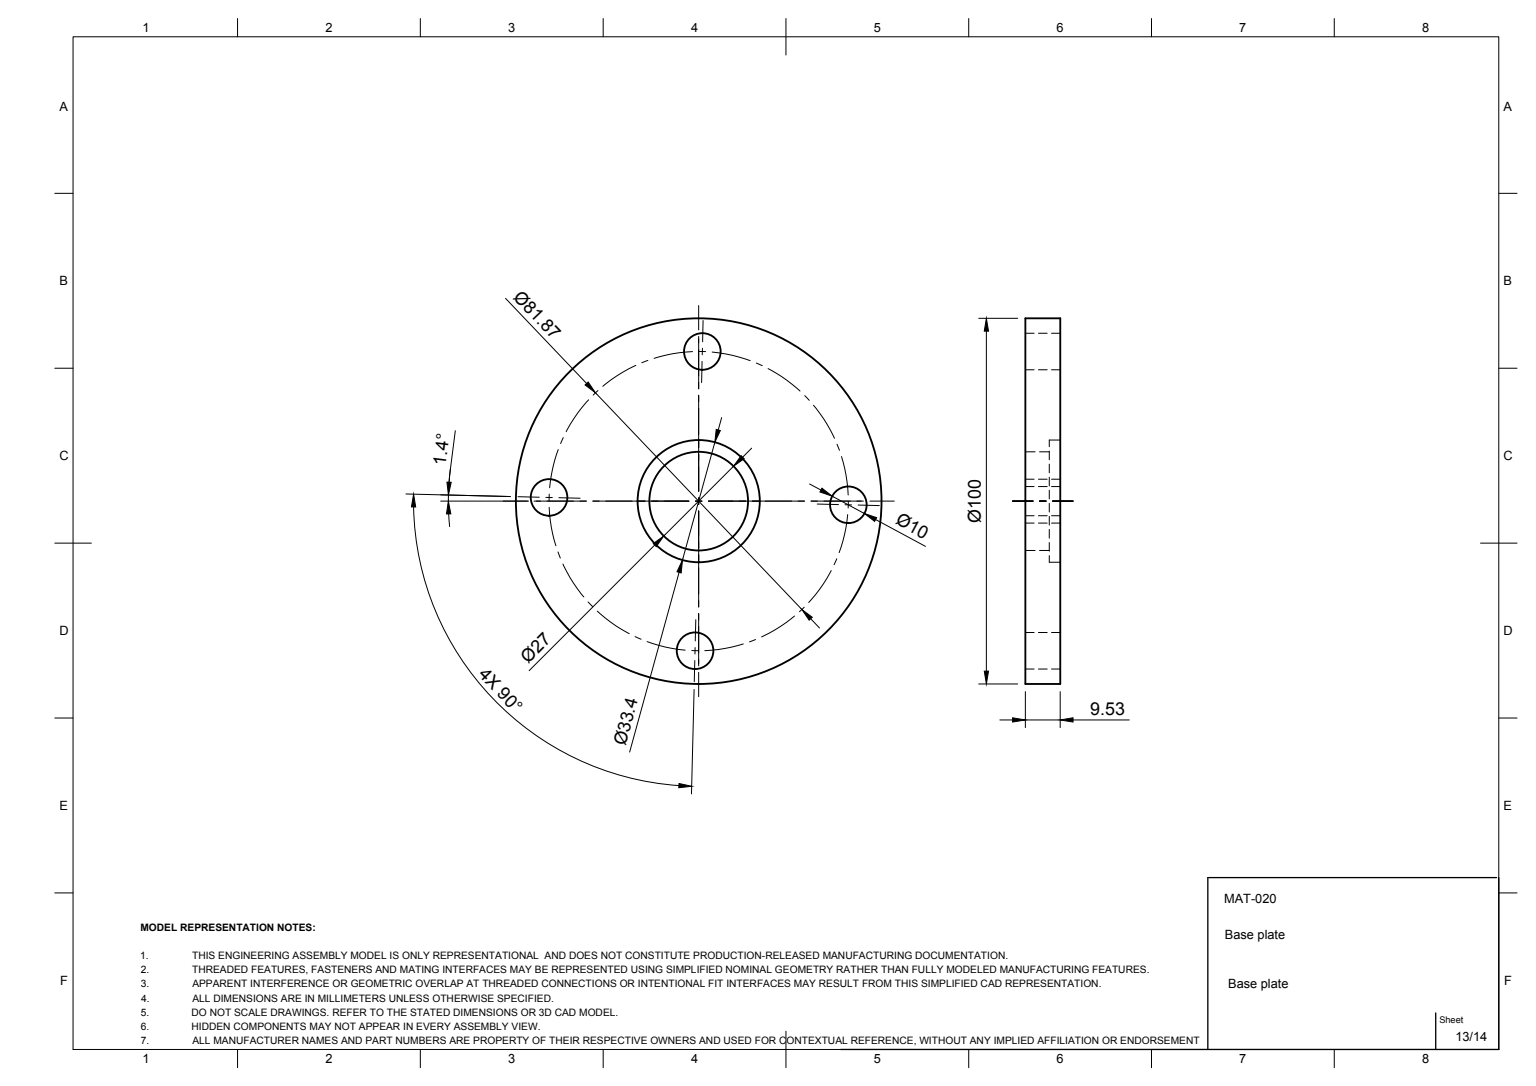
ISO-10303-21;
HEADER;
/* Generated by software containing ST-Developer
 * from STEP Tools, Inc. (www.steptools.com) 
 */

FILE_DESCRIPTION(
/* description */ ('STEP AP214'),
/* implementation_level */ '2;1');

FILE_NAME(
/* name */ 'Base Plate.step',
/* time_stamp */ '2026-11-14T06:20:50-08:00',
/* author */ (''),
/* organization */ (''),
/* preprocessor_version */ 'ST-DEVELOPER v20.2',
/* originating_system */ 'Autodesk Translation Framework v15.17.0.0',
/* authorisation */ '');

FILE_SCHEMA (('AUTOMOTIVE_DESIGN { 1 0 10303 214 3 1 1 }'));
ENDSEC;

DATA;
#10=MECHANICAL_DESIGN_GEOMETRIC_PRESENTATION_REPRESENTATION('',(#964),#20658);
#136=FACE_BOUND('',#1366,.T.);
#137=FACE_BOUND('',#1367,.T.);
#138=FACE_BOUND('',#1368,.T.);
#139=FACE_BOUND('',#1369,.T.);
#140=FACE_BOUND('',#1370,.T.);
#141=FACE_BOUND('',#1372,.T.);
#142=FACE_BOUND('',#1373,.T.);
#143=FACE_BOUND('',#1374,.T.);
#144=FACE_BOUND('',#1375,.T.);
#145=FACE_BOUND('',#1376,.T.);
#146=FACE_BOUND('',#1378,.T.);
#428=PLANE('',#4012);
#429=PLANE('',#4013);
#430=PLANE('',#4014);
#597=LINE('',#20343,#790);
#598=LINE('',#20349,#791);
#599=LINE('',#20355,#792);
#600=LINE('',#20361,#793);
#601=LINE('',#20367,#794);
#602=LINE('',#20373,#795);
#603=LINE('',#20379,#796);
#790=VECTOR('',#4672,13.5);
#791=VECTOR('',#4679,16.7);
#792=VECTOR('',#4686,5.);
#793=VECTOR('',#4693,5.);
#794=VECTOR('',#4700,5.);
#795=VECTOR('',#4707,5.);
#796=VECTOR('',#4714,50.);
#910=CYLINDRICAL_SURFACE('',#3991,13.5);
#911=CYLINDRICAL_SURFACE('',#3994,16.7);
#912=CYLINDRICAL_SURFACE('',#3997,5.);
#913=CYLINDRICAL_SURFACE('',#4000,5.);
#914=CYLINDRICAL_SURFACE('',#4003,5.);
#915=CYLINDRICAL_SURFACE('',#4006,5.);
#916=CYLINDRICAL_SURFACE('',#4009,50.);
#940=SHAPE_REPRESENTATION_RELATIONSHIP('SRR','None',#20724,#952);
#952=ADVANCED_BREP_SHAPE_REPRESENTATION('',(#976),#20654);
#964=STYLED_ITEM('',(#20788),#976);
#976=MANIFOLD_SOLID_BREP('Body1',#3659);
#1137=FACE_OUTER_BOUND('',#1358,.T.);
#1138=FACE_OUTER_BOUND('',#1359,.T.);
#1139=FACE_OUTER_BOUND('',#1360,.T.);
#1140=FACE_OUTER_BOUND('',#1361,.T.);
#1141=FACE_OUTER_BOUND('',#1362,.T.);
#1142=FACE_OUTER_BOUND('',#1363,.T.);
#1143=FACE_OUTER_BOUND('',#1364,.T.);
#1144=FACE_OUTER_BOUND('',#1365,.T.);
#1145=FACE_OUTER_BOUND('',#1371,.T.);
#1146=FACE_OUTER_BOUND('',#1377,.T.);
#1358=EDGE_LOOP('',(#3230,#3231,#3232,#3233));
#1359=EDGE_LOOP('',(#3234,#3235,#3236,#3237));
#1360=EDGE_LOOP('',(#3238,#3239,#3240,#3241));
#1361=EDGE_LOOP('',(#3242,#3243,#3244,#3245));
#1362=EDGE_LOOP('',(#3246,#3247,#3248,#3249));
#1363=EDGE_LOOP('',(#3250,#3251,#3252,#3253));
#1364=EDGE_LOOP('',(#3254,#3255,#3256,#3257));
#1365=EDGE_LOOP('',(#3258));
#1366=EDGE_LOOP('',(#3259));
#1367=EDGE_LOOP('',(#3260));
#1368=EDGE_LOOP('',(#3261));
#1369=EDGE_LOOP('',(#3262));
#1370=EDGE_LOOP('',(#3263));
#1371=EDGE_LOOP('',(#3264));
#1372=EDGE_LOOP('',(#3265));
#1373=EDGE_LOOP('',(#3266));
#1374=EDGE_LOOP('',(#3267));
#1375=EDGE_LOOP('',(#3268));
#1376=EDGE_LOOP('',(#3269));
#1377=EDGE_LOOP('',(#3270));
#1378=EDGE_LOOP('',(#3271));
#1493=CIRCLE('',#3992,13.5);
#1494=CIRCLE('',#3993,13.5);
#1495=CIRCLE('',#3995,16.7);
#1496=CIRCLE('',#3996,16.7);
#1497=CIRCLE('',#3998,5.);
#1498=CIRCLE('',#3999,5.);
#1499=CIRCLE('',#4001,5.);
#1500=CIRCLE('',#4002,5.);
#1501=CIRCLE('',#4004,5.);
#1502=CIRCLE('',#4005,5.);
#1503=CIRCLE('',#4007,5.);
#1504=CIRCLE('',#4008,5.);
#1505=CIRCLE('',#4010,50.);
#1506=CIRCLE('',#4011,50.);
#1821=VERTEX_POINT('',#20340);
#1822=VERTEX_POINT('',#20342);
#1823=VERTEX_POINT('',#20346);
#1824=VERTEX_POINT('',#20348);
#1825=VERTEX_POINT('',#20352);
#1826=VERTEX_POINT('',#20354);
#1827=VERTEX_POINT('',#20358);
#1828=VERTEX_POINT('',#20360);
#1829=VERTEX_POINT('',#20364);
#1830=VERTEX_POINT('',#20366);
#1831=VERTEX_POINT('',#20370);
#1832=VERTEX_POINT('',#20372);
#1833=VERTEX_POINT('',#20376);
#1834=VERTEX_POINT('',#20378);
#2297=EDGE_CURVE('',#1821,#1821,#1493,.T.);
#2298=EDGE_CURVE('',#1821,#1822,#597,.T.);
#2299=EDGE_CURVE('',#1822,#1822,#1494,.T.);
#2300=EDGE_CURVE('',#1823,#1823,#1495,.T.);
#2301=EDGE_CURVE('',#1823,#1824,#598,.T.);
#2302=EDGE_CURVE('',#1824,#1824,#1496,.T.);
#2303=EDGE_CURVE('',#1825,#1825,#1497,.T.);
#2304=EDGE_CURVE('',#1825,#1826,#599,.T.);
#2305=EDGE_CURVE('',#1826,#1826,#1498,.T.);
#2306=EDGE_CURVE('',#1827,#1827,#1499,.T.);
#2307=EDGE_CURVE('',#1827,#1828,#600,.T.);
#2308=EDGE_CURVE('',#1828,#1828,#1500,.T.);
#2309=EDGE_CURVE('',#1829,#1829,#1501,.T.);
#2310=EDGE_CURVE('',#1829,#1830,#601,.T.);
#2311=EDGE_CURVE('',#1830,#1830,#1502,.T.);
#2312=EDGE_CURVE('',#1831,#1831,#1503,.T.);
#2313=EDGE_CURVE('',#1831,#1832,#602,.T.);
#2314=EDGE_CURVE('',#1832,#1832,#1504,.T.);
#2315=EDGE_CURVE('',#1833,#1833,#1505,.T.);
#2316=EDGE_CURVE('',#1833,#1834,#603,.T.);
#2317=EDGE_CURVE('',#1834,#1834,#1506,.T.);
#3230=ORIENTED_EDGE('',*,*,#2297,.F.);
#3231=ORIENTED_EDGE('',*,*,#2298,.T.);
#3232=ORIENTED_EDGE('',*,*,#2299,.T.);
#3233=ORIENTED_EDGE('',*,*,#2298,.F.);
#3234=ORIENTED_EDGE('',*,*,#2300,.F.);
#3235=ORIENTED_EDGE('',*,*,#2301,.T.);
#3236=ORIENTED_EDGE('',*,*,#2302,.T.);
#3237=ORIENTED_EDGE('',*,*,#2301,.F.);
#3238=ORIENTED_EDGE('',*,*,#2303,.T.);
#3239=ORIENTED_EDGE('',*,*,#2304,.T.);
#3240=ORIENTED_EDGE('',*,*,#2305,.F.);
#3241=ORIENTED_EDGE('',*,*,#2304,.F.);
#3242=ORIENTED_EDGE('',*,*,#2306,.T.);
#3243=ORIENTED_EDGE('',*,*,#2307,.T.);
#3244=ORIENTED_EDGE('',*,*,#2308,.F.);
#3245=ORIENTED_EDGE('',*,*,#2307,.F.);
#3246=ORIENTED_EDGE('',*,*,#2309,.T.);
#3247=ORIENTED_EDGE('',*,*,#2310,.T.);
#3248=ORIENTED_EDGE('',*,*,#2311,.F.);
#3249=ORIENTED_EDGE('',*,*,#2310,.F.);
#3250=ORIENTED_EDGE('',*,*,#2312,.T.);
#3251=ORIENTED_EDGE('',*,*,#2313,.T.);
#3252=ORIENTED_EDGE('',*,*,#2314,.F.);
#3253=ORIENTED_EDGE('',*,*,#2313,.F.);
#3254=ORIENTED_EDGE('',*,*,#2315,.T.);
#3255=ORIENTED_EDGE('',*,*,#2316,.T.);
#3256=ORIENTED_EDGE('',*,*,#2317,.F.);
#3257=ORIENTED_EDGE('',*,*,#2316,.F.);
#3258=ORIENTED_EDGE('',*,*,#2317,.T.);
#3259=ORIENTED_EDGE('',*,*,#2309,.F.);
#3260=ORIENTED_EDGE('',*,*,#2303,.F.);
#3261=ORIENTED_EDGE('',*,*,#2302,.F.);
#3262=ORIENTED_EDGE('',*,*,#2306,.F.);
#3263=ORIENTED_EDGE('',*,*,#2312,.F.);
#3264=ORIENTED_EDGE('',*,*,#2315,.F.);
#3265=ORIENTED_EDGE('',*,*,#2314,.T.);
#3266=ORIENTED_EDGE('',*,*,#2311,.T.);
#3267=ORIENTED_EDGE('',*,*,#2308,.T.);
#3268=ORIENTED_EDGE('',*,*,#2305,.T.);
#3269=ORIENTED_EDGE('',*,*,#2297,.T.);
#3270=ORIENTED_EDGE('',*,*,#2300,.T.);
#3271=ORIENTED_EDGE('',*,*,#2299,.F.);
#3599=ADVANCED_FACE('',(#1137),#910,.F.);
#3600=ADVANCED_FACE('',(#1138),#911,.F.);
#3601=ADVANCED_FACE('',(#1139),#912,.F.);
#3602=ADVANCED_FACE('',(#1140),#913,.F.);
#3603=ADVANCED_FACE('',(#1141),#914,.F.);
#3604=ADVANCED_FACE('',(#1142),#915,.F.);
#3605=ADVANCED_FACE('',(#1143),#916,.T.);
#3606=ADVANCED_FACE('',(#1144,#136,#137,#138,#139,#140),#428,.T.);
#3607=ADVANCED_FACE('',(#1145,#141,#142,#143,#144,#145),#429,.F.);
#3608=ADVANCED_FACE('',(#1146,#146),#430,.T.);
#3659=CLOSED_SHELL('',(#3599,#3600,#3601,#3602,#3603,#3604,#3605,#3606,
#3607,#3608));
#3990=AXIS2_PLACEMENT_3D('',#20338,#4666,#4667);
#3991=AXIS2_PLACEMENT_3D('',#20339,#4668,#4669);
#3992=AXIS2_PLACEMENT_3D('',#20341,#4670,#4671);
#3993=AXIS2_PLACEMENT_3D('',#20344,#4673,#4674);
#3994=AXIS2_PLACEMENT_3D('',#20345,#4675,#4676);
#3995=AXIS2_PLACEMENT_3D('',#20347,#4677,#4678);
#3996=AXIS2_PLACEMENT_3D('',#20350,#4680,#4681);
#3997=AXIS2_PLACEMENT_3D('',#20351,#4682,#4683);
#3998=AXIS2_PLACEMENT_3D('',#20353,#4684,#4685);
#3999=AXIS2_PLACEMENT_3D('',#20356,#4687,#4688);
#4000=AXIS2_PLACEMENT_3D('',#20357,#4689,#4690);
#4001=AXIS2_PLACEMENT_3D('',#20359,#4691,#4692);
#4002=AXIS2_PLACEMENT_3D('',#20362,#4694,#4695);
#4003=AXIS2_PLACEMENT_3D('',#20363,#4696,#4697);
#4004=AXIS2_PLACEMENT_3D('',#20365,#4698,#4699);
#4005=AXIS2_PLACEMENT_3D('',#20368,#4701,#4702);
#4006=AXIS2_PLACEMENT_3D('',#20369,#4703,#4704);
#4007=AXIS2_PLACEMENT_3D('',#20371,#4705,#4706);
#4008=AXIS2_PLACEMENT_3D('',#20374,#4708,#4709);
#4009=AXIS2_PLACEMENT_3D('',#20375,#4710,#4711);
#4010=AXIS2_PLACEMENT_3D('',#20377,#4712,#4713);
#4011=AXIS2_PLACEMENT_3D('',#20380,#4715,#4716);
#4012=AXIS2_PLACEMENT_3D('',#20381,#4717,#4718);
#4013=AXIS2_PLACEMENT_3D('',#20382,#4719,#4720);
#4014=AXIS2_PLACEMENT_3D('',#20383,#4721,#4722);
#4666=DIRECTION('axis',(0.,0.,1.));
#4667=DIRECTION('refdir',(1.,0.,0.));
#4668=DIRECTION('center_axis',(0.,1.,0.));
#4669=DIRECTION('ref_axis',(0.,0.,1.));
#4670=DIRECTION('center_axis',(0.,1.,0.));
#4671=DIRECTION('ref_axis',(0.,0.,1.));
#4672=DIRECTION('',(0.,1.,0.));
#4673=DIRECTION('center_axis',(0.,1.,0.));
#4674=DIRECTION('ref_axis',(0.,0.,1.));
#4675=DIRECTION('center_axis',(0.,1.,0.));
#4676=DIRECTION('ref_axis',(0.,0.,1.));
#4677=DIRECTION('center_axis',(0.,1.,0.));
#4678=DIRECTION('ref_axis',(0.,0.,1.));
#4679=DIRECTION('',(0.,1.,0.));
#4680=DIRECTION('center_axis',(0.,1.,0.));
#4681=DIRECTION('ref_axis',(0.,0.,1.));
#4682=DIRECTION('center_axis',(0.,-1.,0.));
#4683=DIRECTION('ref_axis',(0.,0.,-1.));
#4684=DIRECTION('center_axis',(0.,1.,0.));
#4685=DIRECTION('ref_axis',(0.,0.,1.));
#4686=DIRECTION('',(0.,-1.,0.));
#4687=DIRECTION('center_axis',(0.,1.,0.));
#4688=DIRECTION('ref_axis',(0.,0.,1.));
#4689=DIRECTION('center_axis',(0.,-1.,0.));
#4690=DIRECTION('ref_axis',(0.,0.,-1.));
#4691=DIRECTION('center_axis',(0.,1.,0.));
#4692=DIRECTION('ref_axis',(0.,0.,1.));
#4693=DIRECTION('',(0.,-1.,0.));
#4694=DIRECTION('center_axis',(0.,1.,0.));
#4695=DIRECTION('ref_axis',(0.,0.,1.));
#4696=DIRECTION('center_axis',(0.,-1.,0.));
#4697=DIRECTION('ref_axis',(0.,0.,-1.));
#4698=DIRECTION('center_axis',(0.,1.,0.));
#4699=DIRECTION('ref_axis',(0.,0.,1.));
#4700=DIRECTION('',(0.,-1.,0.));
#4701=DIRECTION('center_axis',(0.,1.,0.));
#4702=DIRECTION('ref_axis',(0.,0.,1.));
#4703=DIRECTION('center_axis',(0.,-1.,0.));
#4704=DIRECTION('ref_axis',(0.,0.,-1.));
#4705=DIRECTION('center_axis',(0.,1.,0.));
#4706=DIRECTION('ref_axis',(0.,0.,1.));
#4707=DIRECTION('',(0.,-1.,0.));
#4708=DIRECTION('center_axis',(0.,1.,0.));
#4709=DIRECTION('ref_axis',(0.,0.,1.));
#4710=DIRECTION('center_axis',(0.,-1.,0.));
#4711=DIRECTION('ref_axis',(0.,0.,-1.));
#4712=DIRECTION('center_axis',(0.,1.,0.));
#4713=DIRECTION('ref_axis',(0.,0.,1.));
#4714=DIRECTION('',(0.,1.,0.));
#4715=DIRECTION('center_axis',(0.,1.,0.));
#4716=DIRECTION('ref_axis',(0.,0.,1.));
#4717=DIRECTION('center_axis',(0.,1.,0.));
#4718=DIRECTION('ref_axis',(0.,0.,1.));
#4719=DIRECTION('center_axis',(0.,1.,0.));
#4720=DIRECTION('ref_axis',(0.,0.,1.));
#4721=DIRECTION('center_axis',(0.,1.,0.));
#4722=DIRECTION('ref_axis',(0.,0.,1.));
#20338=CARTESIAN_POINT('',(0.,0.,0.));
#20339=CARTESIAN_POINT('Origin',(0.,-13.475,0.));
#20340=CARTESIAN_POINT('',(-1.65327317884893E-15,0.,-13.5));
#20341=CARTESIAN_POINT('Origin',(0.,0.,0.));
#20342=CARTESIAN_POINT('',(-1.65327317884893E-15,6.525,-13.5));
#20343=CARTESIAN_POINT('',(-1.65327317884893E-15,-13.475,-13.5));
#20344=CARTESIAN_POINT('Origin',(0.,6.525,0.));
#20345=CARTESIAN_POINT('Origin',(0.,6.525,0.));
#20346=CARTESIAN_POINT('',(-2.04516015457608E-15,6.525,-16.7));
#20347=CARTESIAN_POINT('Origin',(0.,6.525,0.));
#20348=CARTESIAN_POINT('',(-2.04516015457608E-15,9.525,-16.7));
#20349=CARTESIAN_POINT('',(-2.04516015457608E-15,6.525,-16.7));
#20350=CARTESIAN_POINT('Origin',(0.,9.525,0.));
#20351=CARTESIAN_POINT('Origin',(-40.9338792388751,9.525,1.85445089342754E-12));
#20352=CARTESIAN_POINT('',(-40.9338792388751,9.525,5.00000000000185));
#20353=CARTESIAN_POINT('Origin',(-40.9338792388751,9.525,1.85445089342754E-12));
#20354=CARTESIAN_POINT('',(-40.9338792388751,0.,5.00000000000185));
#20355=CARTESIAN_POINT('',(-40.9338792388751,9.525,5.00000000000185));
#20356=CARTESIAN_POINT('Origin',(-40.9338792388751,0.,1.85445089342754E-12));
#20357=CARTESIAN_POINT('Origin',(3.69887587801777E-12,9.525,40.9338792388769));
#20358=CARTESIAN_POINT('',(3.6982635546182E-12,9.525,45.9338792388769));
#20359=CARTESIAN_POINT('Origin',(3.69887587801777E-12,9.525,40.9338792388769));
#20360=CARTESIAN_POINT('',(3.6982635546182E-12,0.,45.9338792388769));
#20361=CARTESIAN_POINT('',(3.6982635546182E-12,9.525,45.9338792388769));
#20362=CARTESIAN_POINT('Origin',(3.69887587801777E-12,0.,40.9338792388769));
#20363=CARTESIAN_POINT('Origin',(40.9338792388788,9.525,-1.84943793900889E-12));
#20364=CARTESIAN_POINT('',(40.9338792388788,9.525,4.99999999999815));
#20365=CARTESIAN_POINT('Origin',(40.9338792388788,9.525,-1.84943793900889E-12));
#20366=CARTESIAN_POINT('',(40.9338792388788,0.,4.99999999999815));
#20367=CARTESIAN_POINT('',(40.9338792388788,9.525,4.99999999999815));
#20368=CARTESIAN_POINT('Origin',(40.9338792388788,0.,-1.84943793900889E-12));
#20369=CARTESIAN_POINT('Origin',(0.,9.525,-40.9338792388769));
#20370=CARTESIAN_POINT('',(-6.12323399573676E-16,9.525,-35.9338792388769));
#20371=CARTESIAN_POINT('Origin',(0.,9.525,-40.9338792388769));
#20372=CARTESIAN_POINT('',(-6.12323399573676E-16,0.,-35.9338792388769));
#20373=CARTESIAN_POINT('',(-6.12323399573676E-16,9.525,-35.9338792388769));
#20374=CARTESIAN_POINT('Origin',(0.,0.,-40.9338792388769));
#20375=CARTESIAN_POINT('Origin',(0.,9.525,0.));
#20376=CARTESIAN_POINT('',(-6.12323399573677E-15,0.,50.));
#20377=CARTESIAN_POINT('Origin',(0.,0.,0.));
#20378=CARTESIAN_POINT('',(-6.12323399573677E-15,9.525,50.));
#20379=CARTESIAN_POINT('',(-6.12323399573677E-15,9.525,50.));
#20380=CARTESIAN_POINT('Origin',(0.,9.525,0.));
#20381=CARTESIAN_POINT('Origin',(0.,9.525,0.));
#20382=CARTESIAN_POINT('Origin',(0.,0.,0.));
#20383=CARTESIAN_POINT('Origin',(0.,6.525,0.));
#20640=UNCERTAINTY_MEASURE_WITH_UNIT(LENGTH_MEASURE(0.01),#20659,
'DISTANCE_ACCURACY_VALUE',
'Maximum model space distance between geometric entities at asserted c
onnectivities');
#20644=UNCERTAINTY_MEASURE_WITH_UNIT(LENGTH_MEASURE(0.01),#20659,
'DISTANCE_ACCURACY_VALUE',
'Maximum model space distance between geometric entities at asserted c
onnectivities');
#20654=(
GEOMETRIC_REPRESENTATION_CONTEXT(3)
GLOBAL_UNCERTAINTY_ASSIGNED_CONTEXT((#20640))
GLOBAL_UNIT_ASSIGNED_CONTEXT((#20659,#20661,#20662))
REPRESENTATION_CONTEXT('','3D')
);
#20658=(
GEOMETRIC_REPRESENTATION_CONTEXT(3)
GLOBAL_UNCERTAINTY_ASSIGNED_CONTEXT((#20644))
GLOBAL_UNIT_ASSIGNED_CONTEXT((#20659,#20661,#20662))
REPRESENTATION_CONTEXT('','3D')
);
#20659=(
LENGTH_UNIT()
NAMED_UNIT(*)
SI_UNIT(.MILLI.,.METRE.)
);
#20661=(
NAMED_UNIT(*)
PLANE_ANGLE_UNIT()
SI_UNIT($,.RADIAN.)
);
#20662=(
NAMED_UNIT(*)
SI_UNIT($,.STERADIAN.)
SOLID_ANGLE_UNIT()
);
#20672=SHAPE_DEFINITION_REPRESENTATION(#20685,#20724);
#20685=PRODUCT_DEFINITION_SHAPE('',$,#20738);
#20724=SHAPE_REPRESENTATION('',(#3990),#20654);
#20728=PRODUCT_DEFINITION_CONTEXT('part definition',#20769,'design');
#20738=PRODUCT_DEFINITION('Base plate','Base Plate',#20751,#20728);
#20751=PRODUCT_DEFINITION_FORMATION('',$,#20780);
#20769=APPLICATION_CONTEXT(
'Core Data for Automotive Mechanical Design Process');
#20770=PRODUCT_CONTEXT('part definition',#20769,'mechanical');
#20780=PRODUCT('Base plate','Base Plate','Base plate',(#20770));
#20788=PRESENTATION_STYLE_ASSIGNMENT((#20793));
#20793=SURFACE_STYLE_USAGE(.BOTH.,#20798);
#20798=SURFACE_SIDE_STYLE('',(#20803));
#20803=SURFACE_STYLE_FILL_AREA(#20808);
#20808=FILL_AREA_STYLE('Opaque(20,51,87)',(#20813));
#20813=FILL_AREA_STYLE_COLOUR('Opaque(20,51,87)',#20818);
#20818=COLOUR_RGB('Opaque(20,51,87)',0.0784313725490196,0.2,0.341176470588235);
ENDSEC;
END-ISO-10303-21;
